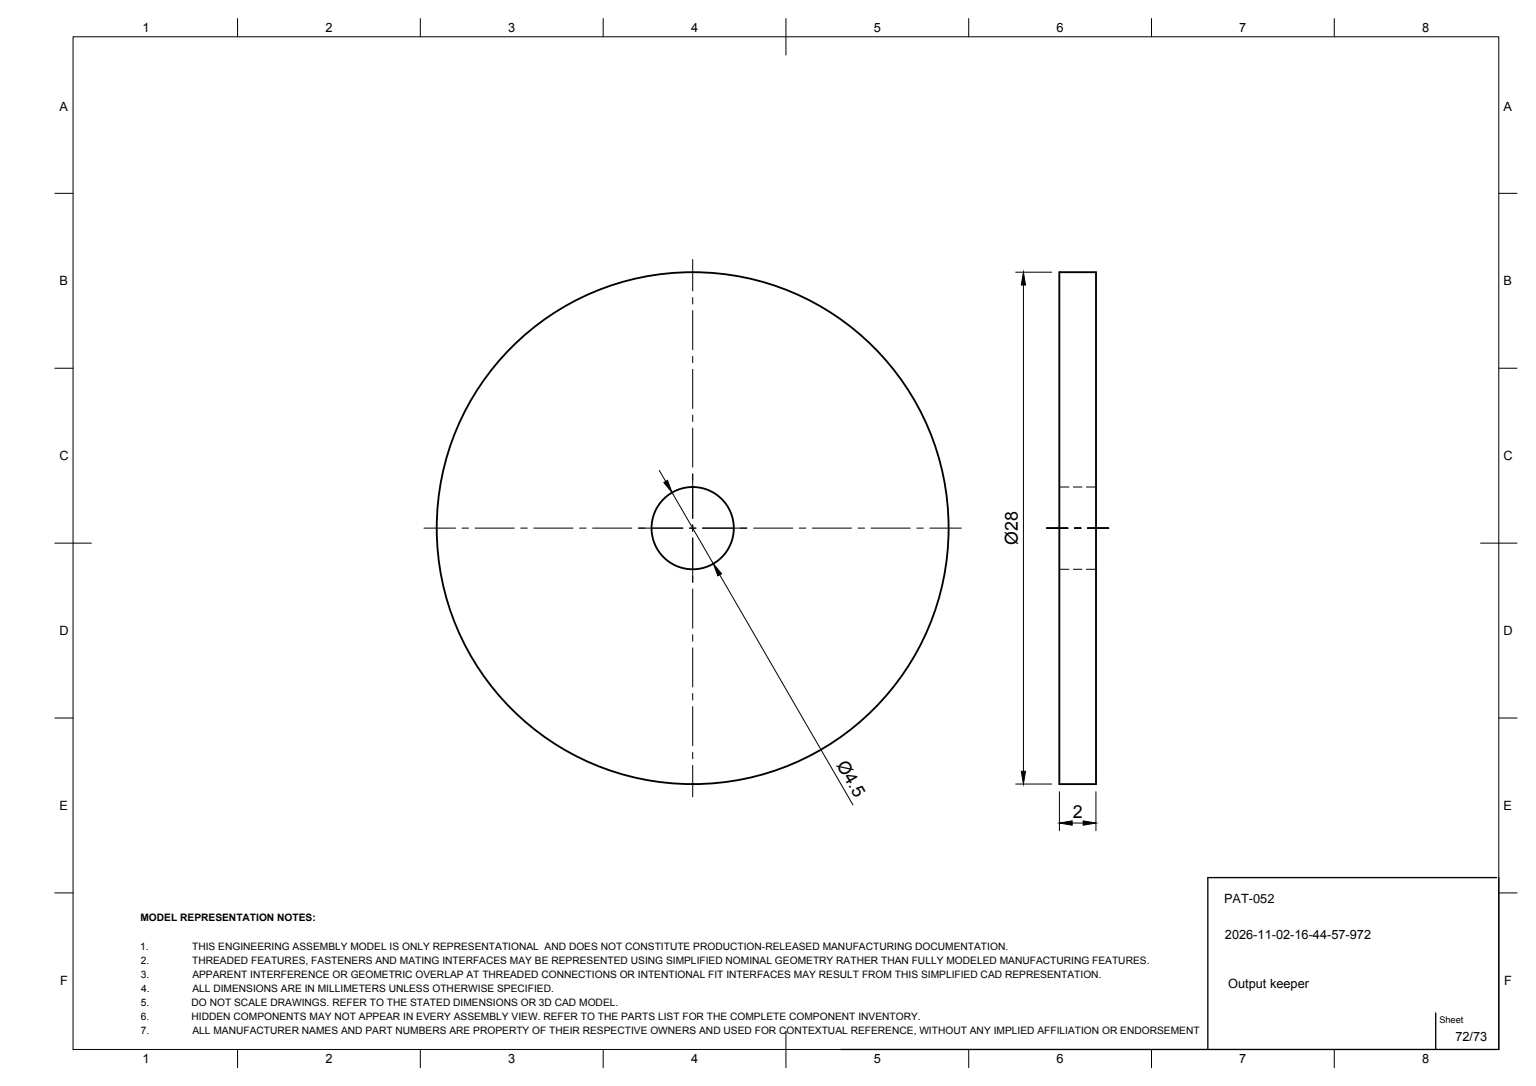
ISO-10303-21;
HEADER;
/* Generated by software containing ST-Developer
 * from STEP Tools, Inc. (www.steptools.com) 
 */

FILE_DESCRIPTION(
/* description */ ('Hand-crank gear train demonstrator'),
/* implementation_level */ '2;1');

FILE_NAME(
/* name */ 'Output keeper.step',
/* time_stamp */ '2026-10-28T03:22:13-07:00',
/* author */ (''),
/* organization */ (''),
/* preprocessor_version */ 'ST-DEVELOPER v20.2',
/* originating_system */ 'Autodesk Translation Framework v15.17.0.0',
/* authorisation */ '');

FILE_SCHEMA (('AUTOMOTIVE_DESIGN { 1 0 10303 214 3 1 1 }'));
ENDSEC;

DATA;
#10=MECHANICAL_DESIGN_GEOMETRIC_PRESENTATION_REPRESENTATION('',(#1262),#62758);
#1119=SHAPE_REPRESENTATION_RELATIONSHIP('SRR','None',#63097,#1183);
#1183=ADVANCED_BREP_SHAPE_REPRESENTATION('',(#1337),#62751);
#1262=STYLED_ITEM('',(#63476),#1337);
#1337=MANIFOLD_SOLID_BREP('Body1',#16446);
#1624=FACE_BOUND('',#4065,.T.);
#1625=FACE_BOUND('',#4067,.T.);
#2043=PLANE('',#18480);
#2044=PLANE('',#18481);
#2844=FACE_OUTER_BOUND('',#4062,.T.);
#2845=FACE_OUTER_BOUND('',#4063,.T.);
#2846=FACE_OUTER_BOUND('',#4064,.T.);
#2847=FACE_OUTER_BOUND('',#4066,.T.);
#4062=EDGE_LOOP('',(#13991,#13992,#13993,#13994));
#4063=EDGE_LOOP('',(#13995,#13996,#13997,#13998));
#4064=EDGE_LOOP('',(#13999));
#4065=EDGE_LOOP('',(#14000));
#4066=EDGE_LOOP('',(#14001));
#4067=EDGE_LOOP('',(#14002));
#5174=LINE('',#38744,#6306);
#5175=LINE('',#38750,#6307);
#6306=VECTOR('',#22355,0.225000000000001);
#6307=VECTOR('',#22362,1.4);
#7108=CIRCLE('',#18475,0.225000000000001);
#7109=CIRCLE('',#18476,0.225000000000001);
#7110=CIRCLE('',#18478,1.4);
#7111=CIRCLE('',#18479,1.4);
#8279=VERTEX_POINT('',#38741);
#8280=VERTEX_POINT('',#38743);
#8281=VERTEX_POINT('',#38747);
#8282=VERTEX_POINT('',#38749);
#10247=EDGE_CURVE('',#8279,#8279,#7108,.T.);
#10248=EDGE_CURVE('',#8279,#8280,#5174,.T.);
#10249=EDGE_CURVE('',#8280,#8280,#7109,.T.);
#10250=EDGE_CURVE('',#8281,#8281,#7110,.T.);
#10251=EDGE_CURVE('',#8281,#8282,#5175,.T.);
#10252=EDGE_CURVE('',#8282,#8282,#7111,.T.);
#13991=ORIENTED_EDGE('',*,*,#10247,.F.);
#13992=ORIENTED_EDGE('',*,*,#10248,.T.);
#13993=ORIENTED_EDGE('',*,*,#10249,.T.);
#13994=ORIENTED_EDGE('',*,*,#10248,.F.);
#13995=ORIENTED_EDGE('',*,*,#10250,.F.);
#13996=ORIENTED_EDGE('',*,*,#10251,.T.);
#13997=ORIENTED_EDGE('',*,*,#10252,.T.);
#13998=ORIENTED_EDGE('',*,*,#10251,.F.);
#13999=ORIENTED_EDGE('',*,*,#10250,.T.);
#14000=ORIENTED_EDGE('',*,*,#10247,.T.);
#14001=ORIENTED_EDGE('',*,*,#10252,.F.);
#14002=ORIENTED_EDGE('',*,*,#10249,.F.);
#15384=CYLINDRICAL_SURFACE('',#18474,0.225000000000001);
#15385=CYLINDRICAL_SURFACE('',#18477,1.4);
#16154=ADVANCED_FACE('',(#2844),#15384,.F.);
#16155=ADVANCED_FACE('',(#2845),#15385,.T.);
#16156=ADVANCED_FACE('',(#2846,#1624),#2043,.T.);
#16157=ADVANCED_FACE('',(#2847,#1625),#2044,.F.);
#16446=CLOSED_SHELL('',(#16154,#16155,#16156,#16157));
#18473=AXIS2_PLACEMENT_3D('',#38739,#22349,#22350);
#18474=AXIS2_PLACEMENT_3D('',#38740,#22351,#22352);
#18475=AXIS2_PLACEMENT_3D('',#38742,#22353,#22354);
#18476=AXIS2_PLACEMENT_3D('',#38745,#22356,#22357);
#18477=AXIS2_PLACEMENT_3D('',#38746,#22358,#22359);
#18478=AXIS2_PLACEMENT_3D('',#38748,#22360,#22361);
#18479=AXIS2_PLACEMENT_3D('',#38751,#22363,#22364);
#18480=AXIS2_PLACEMENT_3D('',#38752,#22365,#22366);
#18481=AXIS2_PLACEMENT_3D('',#38753,#22367,#22368);
#22349=DIRECTION('axis',(0.,0.,1.));
#22350=DIRECTION('refdir',(1.,0.,0.));
#22351=DIRECTION('center_axis',(0.,1.,0.));
#22352=DIRECTION('ref_axis',(1.,0.,0.));
#22353=DIRECTION('center_axis',(0.,-1.,0.));
#22354=DIRECTION('ref_axis',(1.,0.,0.));
#22355=DIRECTION('',(0.,-1.,0.));
#22356=DIRECTION('center_axis',(0.,-1.,0.));
#22357=DIRECTION('ref_axis',(1.,0.,0.));
#22358=DIRECTION('center_axis',(0.,1.,0.));
#22359=DIRECTION('ref_axis',(1.,0.,0.));
#22360=DIRECTION('center_axis',(0.,1.,0.));
#22361=DIRECTION('ref_axis',(1.,0.,0.));
#22362=DIRECTION('',(0.,-1.,0.));
#22363=DIRECTION('center_axis',(0.,1.,0.));
#22364=DIRECTION('ref_axis',(1.,0.,0.));
#22365=DIRECTION('center_axis',(0.,1.,0.));
#22366=DIRECTION('ref_axis',(1.,0.,0.));
#22367=DIRECTION('center_axis',(0.,1.,0.));
#22368=DIRECTION('ref_axis',(1.,0.,0.));
#38739=CARTESIAN_POINT('',(0.,0.,0.));
#38740=CARTESIAN_POINT('Origin',(18.,6.,9.));
#38741=CARTESIAN_POINT('',(17.775,6.2,9.));
#38742=CARTESIAN_POINT('Origin',(18.,6.2,9.));
#38743=CARTESIAN_POINT('',(17.775,6.,9.));
#38744=CARTESIAN_POINT('',(17.775,6.,9.));
#38745=CARTESIAN_POINT('Origin',(18.,6.,9.));
#38746=CARTESIAN_POINT('Origin',(18.,6.,9.));
#38747=CARTESIAN_POINT('',(16.6,6.2,9.));
#38748=CARTESIAN_POINT('Origin',(18.,6.2,9.));
#38749=CARTESIAN_POINT('',(16.6,6.,9.));
#38750=CARTESIAN_POINT('',(16.6,6.,9.));
#38751=CARTESIAN_POINT('Origin',(18.,6.,9.));
#38752=CARTESIAN_POINT('Origin',(18.,6.2,9.));
#38753=CARTESIAN_POINT('Origin',(18.,6.,9.));
#62677=UNCERTAINTY_MEASURE_WITH_UNIT(LENGTH_MEASURE(0.001),#62759,
'DISTANCE_ACCURACY_VALUE',
'Maximum model space distance between geometric entities at asserted c
onnectivities');
#62684=UNCERTAINTY_MEASURE_WITH_UNIT(LENGTH_MEASURE(0.001),#62759,
'DISTANCE_ACCURACY_VALUE',
'Maximum model space distance between geometric entities at asserted c
onnectivities');
#62751=(
GEOMETRIC_REPRESENTATION_CONTEXT(3)
GLOBAL_UNCERTAINTY_ASSIGNED_CONTEXT((#62677))
GLOBAL_UNIT_ASSIGNED_CONTEXT((#62759,#62761,#62762))
REPRESENTATION_CONTEXT('','3D')
);
#62758=(
GEOMETRIC_REPRESENTATION_CONTEXT(3)
GLOBAL_UNCERTAINTY_ASSIGNED_CONTEXT((#62684))
GLOBAL_UNIT_ASSIGNED_CONTEXT((#62759,#62761,#62762))
REPRESENTATION_CONTEXT('','3D')
);
#62759=(
LENGTH_UNIT()
NAMED_UNIT(*)
SI_UNIT(.CENTI.,.METRE.)
);
#62761=(
NAMED_UNIT(*)
PLANE_ANGLE_UNIT()
SI_UNIT($,.RADIAN.)
);
#62762=(
NAMED_UNIT(*)
SI_UNIT($,.STERADIAN.)
SOLID_ANGLE_UNIT()
);
#62829=SHAPE_DEFINITION_REPRESENTATION(#62912,#63097);
#62912=PRODUCT_DEFINITION_SHAPE('',$,#63171);
#63097=SHAPE_REPRESENTATION('',(#18473),#62751);
#63104=PRODUCT_DEFINITION_CONTEXT('part definition',#63325,'design');
#63171=PRODUCT_DEFINITION('Output keeper','Output keeper',#63244,#63104);
#63244=PRODUCT_DEFINITION_FORMATION('',$,#63393);
#63325=APPLICATION_CONTEXT(
'Core Data for Automotive Mechanical Design Process');
#63326=PRODUCT_CONTEXT('part definition',#63325,'mechanical');
#63393=PRODUCT('Output keeper','Output keeper','Output keeper',(#63326));
#63470=COLOUR_RGB('Off White',0.89,0.88,0.83);
#63471=FILL_AREA_STYLE_COLOUR('',#63470);
#63472=FILL_AREA_STYLE('',(#63471));
#63473=SURFACE_STYLE_FILL_AREA(#63472);
#63474=SURFACE_SIDE_STYLE('',(#63473));
#63475=SURFACE_STYLE_USAGE(.BOTH.,#63474);
#63476=PRESENTATION_STYLE_ASSIGNMENT((#63475));
ENDSEC;
END-ISO-10303-21;
